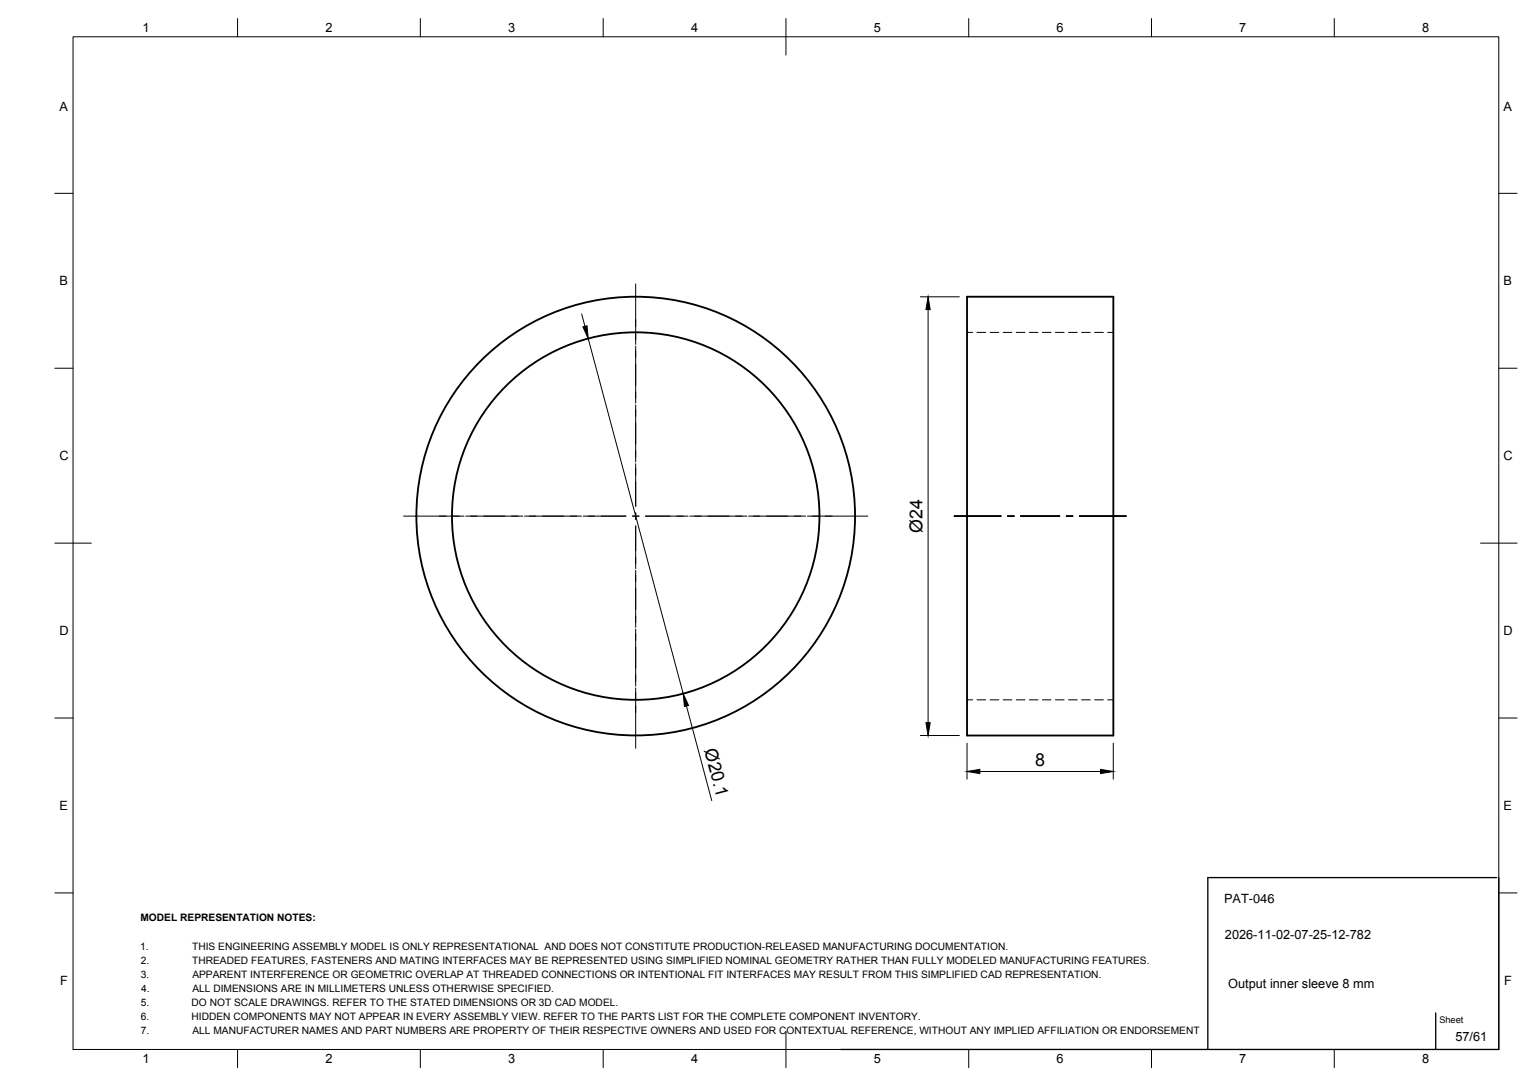
ISO-10303-21;
HEADER;
/* Generated by software containing ST-Developer
 * from STEP Tools, Inc. (www.steptools.com) 
 */

FILE_DESCRIPTION(
/* description */ ('Gear mesh backlash fixture'),
/* implementation_level */ '2;1');

FILE_NAME(
/* name */ 'Output inner sleeve 8 mm.step',
/* time_stamp */ '2026-10-28T03:26:00-07:00',
/* author */ (''),
/* organization */ (''),
/* preprocessor_version */ 'ST-DEVELOPER v20.2',
/* originating_system */ 'Autodesk Translation Framework v15.17.0.0',
/* authorisation */ '');

FILE_SCHEMA (('AUTOMOTIVE_DESIGN { 1 0 10303 214 3 1 1 }'));
ENDSEC;

DATA;
#10=MECHANICAL_DESIGN_GEOMETRIC_PRESENTATION_REPRESENTATION('',(#1074),#57900);
#959=SHAPE_REPRESENTATION_RELATIONSHIP('SRR','None',#58160,#1009);
#1009=ADVANCED_BREP_SHAPE_REPRESENTATION('',(#1137),#57893);
#1074=STYLED_ITEM('',(#58451),#1137);
#1137=MANIFOLD_SOLID_BREP('Body1',#13636);
#1317=FACE_BOUND('',#3187,.T.);
#1318=FACE_BOUND('',#3189,.T.);
#1616=PLANE('',#15263);
#1617=PLANE('',#15264);
#2245=FACE_OUTER_BOUND('',#3184,.T.);
#2246=FACE_OUTER_BOUND('',#3185,.T.);
#2247=FACE_OUTER_BOUND('',#3186,.T.);
#2248=FACE_OUTER_BOUND('',#3188,.T.);
#3184=EDGE_LOOP('',(#11419,#11420,#11421,#11422));
#3185=EDGE_LOOP('',(#11423,#11424,#11425,#11426));
#3186=EDGE_LOOP('',(#11427));
#3187=EDGE_LOOP('',(#11428));
#3188=EDGE_LOOP('',(#11429));
#3189=EDGE_LOOP('',(#11430));
#4067=LINE('',#33893,#4956);
#4068=LINE('',#33899,#4957);
#4956=VECTOR('',#18362,1.005);
#4957=VECTOR('',#18369,1.2);
#5675=CIRCLE('',#15258,1.005);
#5676=CIRCLE('',#15259,1.005);
#5677=CIRCLE('',#15261,1.2);
#5678=CIRCLE('',#15262,1.2);
#6638=VERTEX_POINT('',#33890);
#6639=VERTEX_POINT('',#33892);
#6640=VERTEX_POINT('',#33896);
#6641=VERTEX_POINT('',#33898);
#8296=EDGE_CURVE('',#6638,#6638,#5675,.T.);
#8297=EDGE_CURVE('',#6638,#6639,#4067,.T.);
#8298=EDGE_CURVE('',#6639,#6639,#5676,.T.);
#8299=EDGE_CURVE('',#6640,#6640,#5677,.T.);
#8300=EDGE_CURVE('',#6640,#6641,#4068,.T.);
#8301=EDGE_CURVE('',#6641,#6641,#5678,.T.);
#11419=ORIENTED_EDGE('',*,*,#8296,.F.);
#11420=ORIENTED_EDGE('',*,*,#8297,.T.);
#11421=ORIENTED_EDGE('',*,*,#8298,.T.);
#11422=ORIENTED_EDGE('',*,*,#8297,.F.);
#11423=ORIENTED_EDGE('',*,*,#8299,.F.);
#11424=ORIENTED_EDGE('',*,*,#8300,.T.);
#11425=ORIENTED_EDGE('',*,*,#8301,.T.);
#11426=ORIENTED_EDGE('',*,*,#8300,.F.);
#11427=ORIENTED_EDGE('',*,*,#8299,.T.);
#11428=ORIENTED_EDGE('',*,*,#8296,.T.);
#11429=ORIENTED_EDGE('',*,*,#8301,.F.);
#11430=ORIENTED_EDGE('',*,*,#8298,.F.);
#12759=CYLINDRICAL_SURFACE('',#15257,1.005);
#12760=CYLINDRICAL_SURFACE('',#15260,1.2);
#13362=ADVANCED_FACE('',(#2245),#12759,.F.);
#13363=ADVANCED_FACE('',(#2246),#12760,.T.);
#13364=ADVANCED_FACE('',(#2247,#1317),#1616,.T.);
#13365=ADVANCED_FACE('',(#2248,#1318),#1617,.F.);
#13636=CLOSED_SHELL('',(#13362,#13363,#13364,#13365));
#15256=AXIS2_PLACEMENT_3D('',#33888,#18356,#18357);
#15257=AXIS2_PLACEMENT_3D('',#33889,#18358,#18359);
#15258=AXIS2_PLACEMENT_3D('',#33891,#18360,#18361);
#15259=AXIS2_PLACEMENT_3D('',#33894,#18363,#18364);
#15260=AXIS2_PLACEMENT_3D('',#33895,#18365,#18366);
#15261=AXIS2_PLACEMENT_3D('',#33897,#18367,#18368);
#15262=AXIS2_PLACEMENT_3D('',#33900,#18370,#18371);
#15263=AXIS2_PLACEMENT_3D('',#33901,#18372,#18373);
#15264=AXIS2_PLACEMENT_3D('',#33902,#18374,#18375);
#18356=DIRECTION('axis',(0.,0.,1.));
#18357=DIRECTION('refdir',(1.,0.,0.));
#18358=DIRECTION('center_axis',(0.,0.,1.));
#18359=DIRECTION('ref_axis',(1.,0.,0.));
#18360=DIRECTION('center_axis',(0.,0.,-1.));
#18361=DIRECTION('ref_axis',(1.,0.,0.));
#18362=DIRECTION('',(0.,0.,-1.));
#18363=DIRECTION('center_axis',(0.,0.,-1.));
#18364=DIRECTION('ref_axis',(1.,0.,0.));
#18365=DIRECTION('center_axis',(0.,0.,1.));
#18366=DIRECTION('ref_axis',(1.,0.,0.));
#18367=DIRECTION('center_axis',(0.,0.,1.));
#18368=DIRECTION('ref_axis',(1.,0.,0.));
#18369=DIRECTION('',(0.,0.,-1.));
#18370=DIRECTION('center_axis',(0.,0.,1.));
#18371=DIRECTION('ref_axis',(1.,0.,0.));
#18372=DIRECTION('center_axis',(0.,0.,1.));
#18373=DIRECTION('ref_axis',(1.,0.,0.));
#18374=DIRECTION('center_axis',(0.,0.,1.));
#18375=DIRECTION('ref_axis',(1.,0.,0.));
#33888=CARTESIAN_POINT('',(0.,0.,0.));
#33889=CARTESIAN_POINT('Origin',(6.,0.,14.2));
#33890=CARTESIAN_POINT('',(4.995,-1.23077003314309E-16,15.));
#33891=CARTESIAN_POINT('Origin',(6.,0.,15.));
#33892=CARTESIAN_POINT('',(4.995,-1.23077003314309E-16,14.2));
#33893=CARTESIAN_POINT('',(4.995,-1.23077003314309E-16,14.2));
#33894=CARTESIAN_POINT('Origin',(6.,0.,14.2));
#33895=CARTESIAN_POINT('Origin',(6.,0.,14.2));
#33896=CARTESIAN_POINT('',(4.8,-1.46957615897682E-16,15.));
#33897=CARTESIAN_POINT('Origin',(6.,0.,15.));
#33898=CARTESIAN_POINT('',(4.8,-1.46957615897682E-16,14.2));
#33899=CARTESIAN_POINT('',(4.8,-1.46957615897682E-16,14.2));
#33900=CARTESIAN_POINT('Origin',(6.,0.,14.2));
#33901=CARTESIAN_POINT('Origin',(6.,0.,15.));
#33902=CARTESIAN_POINT('Origin',(6.,0.,14.2));
#57834=UNCERTAINTY_MEASURE_WITH_UNIT(LENGTH_MEASURE(0.001),#57901,
'DISTANCE_ACCURACY_VALUE',
'Maximum model space distance between geometric entities at asserted c
onnectivities');
#57841=UNCERTAINTY_MEASURE_WITH_UNIT(LENGTH_MEASURE(0.001),#57901,
'DISTANCE_ACCURACY_VALUE',
'Maximum model space distance between geometric entities at asserted c
onnectivities');
#57893=(
GEOMETRIC_REPRESENTATION_CONTEXT(3)
GLOBAL_UNCERTAINTY_ASSIGNED_CONTEXT((#57834))
GLOBAL_UNIT_ASSIGNED_CONTEXT((#57901,#57903,#57904))
REPRESENTATION_CONTEXT('','3D')
);
#57900=(
GEOMETRIC_REPRESENTATION_CONTEXT(3)
GLOBAL_UNCERTAINTY_ASSIGNED_CONTEXT((#57841))
GLOBAL_UNIT_ASSIGNED_CONTEXT((#57901,#57903,#57904))
REPRESENTATION_CONTEXT('','3D')
);
#57901=(
LENGTH_UNIT()
NAMED_UNIT(*)
SI_UNIT(.CENTI.,.METRE.)
);
#57903=(
NAMED_UNIT(*)
PLANE_ANGLE_UNIT()
SI_UNIT($,.RADIAN.)
);
#57904=(
NAMED_UNIT(*)
SI_UNIT($,.STERADIAN.)
SOLID_ANGLE_UNIT()
);
#57956=SHAPE_DEFINITION_REPRESENTATION(#58027,#58160);
#58027=PRODUCT_DEFINITION_SHAPE('',$,#58219);
#58160=SHAPE_REPRESENTATION('',(#15256),#57893);
#58167=PRODUCT_DEFINITION_CONTEXT('part definition',#58343,'design');
#58219=PRODUCT_DEFINITION('Output inner sleeve 8 mm',
'Output inner sleeve 8 mm',#58277,#58167);
#58277=PRODUCT_DEFINITION_FORMATION('',$,#58396);
#58343=APPLICATION_CONTEXT(
'Core Data for Automotive Mechanical Design Process');
#58344=PRODUCT_CONTEXT('part definition',#58343,'mechanical');
#58396=PRODUCT('Output inner sleeve 8 mm','Output inner sleeve 8 mm',
'Output inner sleeve 8 mm',(#58344));
#58445=COLOUR_RGB('Light Blue',0.38,0.62,0.78);
#58446=FILL_AREA_STYLE_COLOUR('',#58445);
#58447=FILL_AREA_STYLE('',(#58446));
#58448=SURFACE_STYLE_FILL_AREA(#58447);
#58449=SURFACE_SIDE_STYLE('',(#58448));
#58450=SURFACE_STYLE_USAGE(.BOTH.,#58449);
#58451=PRESENTATION_STYLE_ASSIGNMENT((#58450));
ENDSEC;
END-ISO-10303-21;
